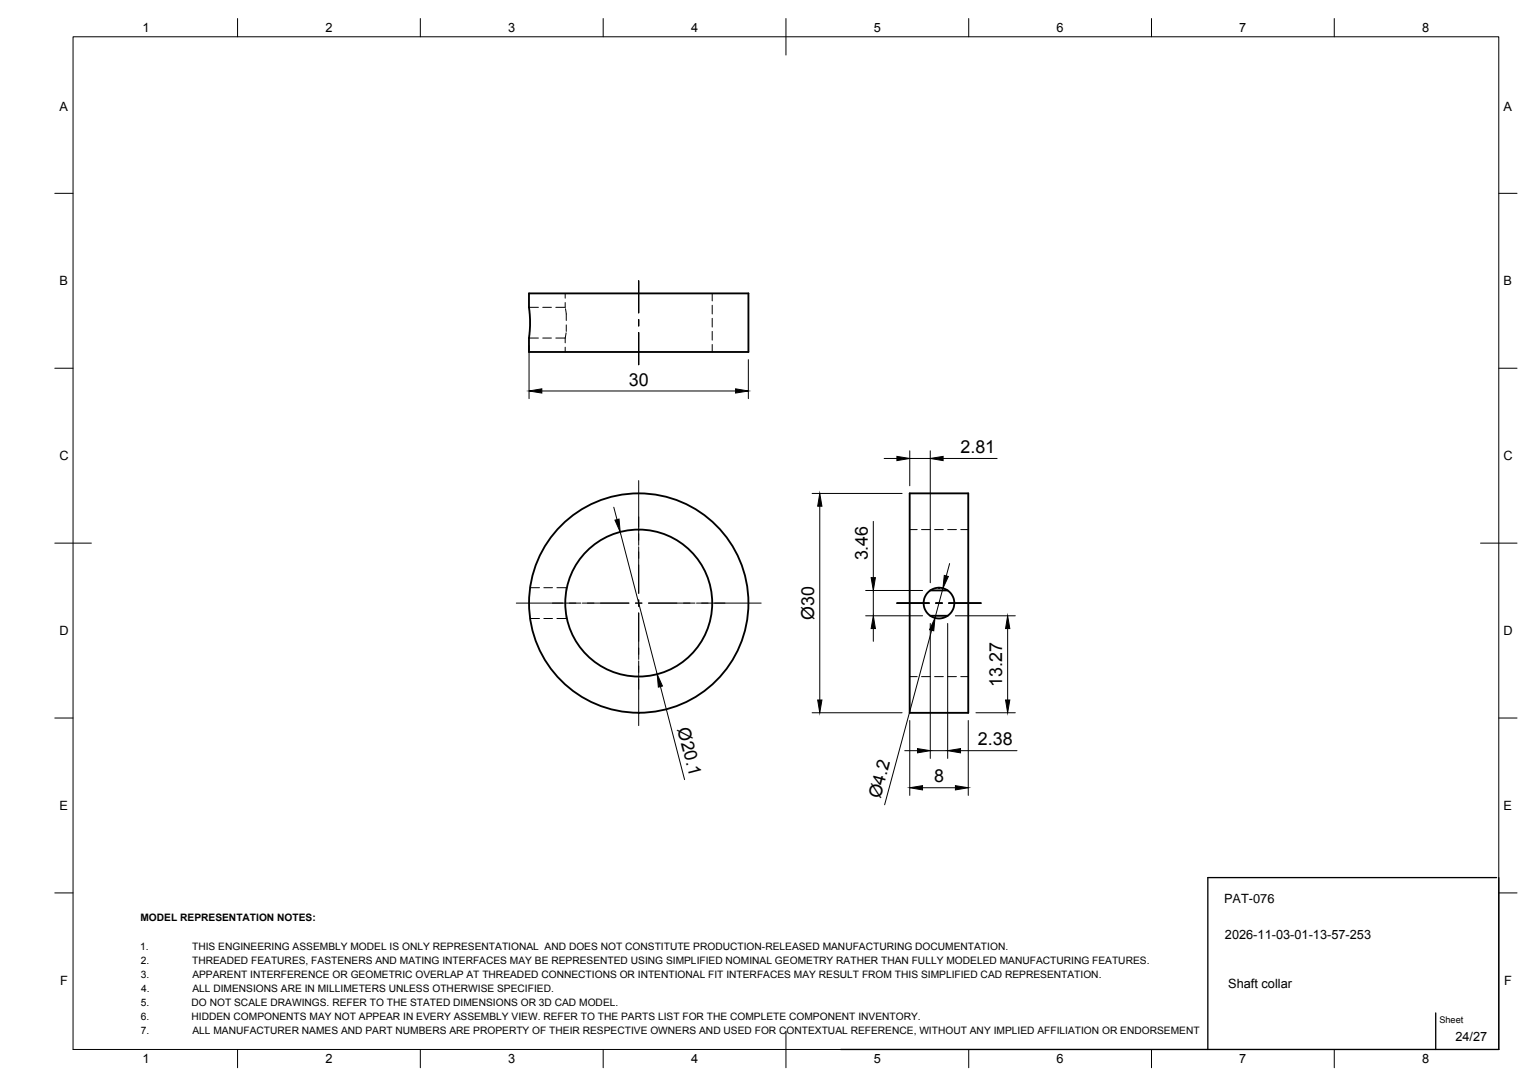
ISO-10303-21;
HEADER;
/* Generated by software containing ST-Developer
 * from STEP Tools, Inc. (www.steptools.com) 
 */

FILE_DESCRIPTION(
/* description */ ('Overhung pulley bearing cartridge'),
/* implementation_level */ '2;1');

FILE_NAME(
/* name */ 'Shaft collar.step',
/* time_stamp */ '2026-10-28T03:22:33-07:00',
/* author */ (''),
/* organization */ (''),
/* preprocessor_version */ 'ST-DEVELOPER v20.2',
/* originating_system */ 'Autodesk Translation Framework v15.17.0.0',
/* authorisation */ '');

FILE_SCHEMA (('AUTOMOTIVE_DESIGN { 1 0 10303 214 3 1 1 }'));
ENDSEC;

DATA;
#10=MECHANICAL_DESIGN_GEOMETRIC_PRESENTATION_REPRESENTATION('',(#308),#10963);
#181=B_SPLINE_CURVE_WITH_KNOTS('',3,(#9804,#9805,#9806,#9807,#9808,#9809,
#9810,#9811,#9812,#9813,#9814,#9815,#9816,#9817),.UNSPECIFIED.,.F.,.F.,
(4,2,2,2,2,2,4),(0.756005737987012,0.793568827564648,0.872922520054202,
0.952276212543757,1.03162990503331,1.11098359752287,1.1485466871005),
 .UNSPECIFIED.);
#182=B_SPLINE_CURVE_WITH_KNOTS('',3,(#9823,#9824,#9825,#9826,#9827,#9828,
#9829,#9830,#9831,#9832,#9833,#9834,#9835,#9836,#9837,#9838,#9839,#9840),
 .UNSPECIFIED.,.F.,.F.,(4,2,2,2,2,2,2,2,4),(0.,0.0792165807733632,0.158433161546726,
0.237648697074571,0.316864232602415,0.396079768130259,0.475295303658103,
0.554511884431466,0.63372846520483),.UNSPECIFIED.);
#183=B_SPLINE_CURVE_WITH_KNOTS('',3,(#9841,#9842,#9843,#9844,#9845,#9846,
#9847,#9848,#9849,#9850,#9851,#9852,#9853,#9854,#9855,#9856,#9857,#9858),
 .UNSPECIFIED.,.F.,.F.,(4,2,2,2,2,2,2,2,4),(0.63372846520483,0.712945045978192,
0.792161626751555,0.8713771622794,0.950592697807244,1.02980823333509,1.10902376886293,
1.1882403496363,1.26745693040966),.UNSPECIFIED.);
#184=B_SPLINE_CURVE_WITH_KNOTS('',3,(#9861,#9862,#9863,#9864,#9865,#9866,
#9867,#9868,#9869,#9870,#9871,#9872,#9873,#9874),.UNSPECIFIED.,.F.,.F.,
(4,2,2,2,2,2,4),(0.121154929624506,0.158718019202143,0.238071711691698,
0.317425404181252,0.396779096670807,0.476132789160362,0.513695878738),
 .UNSPECIFIED.);
#256=SHAPE_REPRESENTATION_RELATIONSHIP('SRR','None',#11078,#278);
#278=ADVANCED_BREP_SHAPE_REPRESENTATION('',(#336),#10958);
#308=STYLED_ITEM('',(#11253),#336);
#336=MANIFOLD_SOLID_BREP('Body1',#5677);
#413=FACE_BOUND('',#1179,.T.);
#414=FACE_BOUND('',#1181,.T.);
#415=FACE_BOUND('',#1183,.T.);
#416=FACE_BOUND('',#1185,.T.);
#542=PLANE('',#6355);
#543=PLANE('',#6360);
#544=PLANE('',#6367);
#545=PLANE('',#6368);
#774=FACE_OUTER_BOUND('',#1175,.T.);
#775=FACE_OUTER_BOUND('',#1176,.T.);
#776=FACE_OUTER_BOUND('',#1177,.T.);
#777=FACE_OUTER_BOUND('',#1178,.T.);
#778=FACE_OUTER_BOUND('',#1180,.T.);
#779=FACE_OUTER_BOUND('',#1182,.T.);
#780=FACE_OUTER_BOUND('',#1184,.T.);
#1175=EDGE_LOOP('',(#4435,#4436));
#1176=EDGE_LOOP('',(#4437,#4438,#4439,#4440,#4441,#4442,#4443,#4444,#4445));
#1177=EDGE_LOOP('',(#4446,#4447,#4448));
#1178=EDGE_LOOP('',(#4449,#4450,#4451,#4452));
#1179=EDGE_LOOP('',(#4453,#4454,#4455,#4456));
#1180=EDGE_LOOP('',(#4457,#4458,#4459,#4460));
#1181=EDGE_LOOP('',(#4461,#4462));
#1182=EDGE_LOOP('',(#4463));
#1183=EDGE_LOOP('',(#4464));
#1184=EDGE_LOOP('',(#4465));
#1185=EDGE_LOOP('',(#4466));
#1517=LINE('',#9800,#1859);
#1518=LINE('',#9821,#1860);
#1519=LINE('',#9876,#1861);
#1520=LINE('',#9881,#1862);
#1521=LINE('',#9887,#1863);
#1859=VECTOR('',#7739,1.);
#1860=VECTOR('',#7746,0.21);
#1861=VECTOR('',#7751,1.);
#1862=VECTOR('',#7756,1.005);
#1863=VECTOR('',#7763,1.5);
#2196=CIRCLE('',#6356,0.21);
#2197=CIRCLE('',#6358,0.21);
#2198=CIRCLE('',#6359,0.21);
#2199=CIRCLE('',#6362,1.005);
#2200=CIRCLE('',#6363,1.005);
#2201=CIRCLE('',#6365,1.5);
#2202=CIRCLE('',#6366,1.5);
#2649=VERTEX_POINT('',#9798);
#2650=VERTEX_POINT('',#9799);
#2651=VERTEX_POINT('',#9803);
#2652=VERTEX_POINT('',#9818);
#2653=VERTEX_POINT('',#9820);
#2654=VERTEX_POINT('',#9822);
#2655=VERTEX_POINT('',#9859);
#2656=VERTEX_POINT('',#9878);
#2657=VERTEX_POINT('',#9880);
#2658=VERTEX_POINT('',#9884);
#2659=VERTEX_POINT('',#9886);
#3287=EDGE_CURVE('',#2649,#2650,#1517,.T.);
#3288=EDGE_CURVE('',#2649,#2650,#2196,.T.);
#3289=EDGE_CURVE('',#2651,#2649,#181,.T.);
#3290=EDGE_CURVE('',#2652,#2651,#2197,.T.);
#3291=EDGE_CURVE('',#2652,#2653,#1518,.T.);
#3292=EDGE_CURVE('',#2654,#2653,#182,.T.);
#3293=EDGE_CURVE('',#2653,#2654,#183,.T.);
#3294=EDGE_CURVE('',#2655,#2652,#2198,.T.);
#3295=EDGE_CURVE('',#2650,#2655,#184,.T.);
#3296=EDGE_CURVE('',#2655,#2651,#1519,.T.);
#3297=EDGE_CURVE('',#2656,#2656,#2199,.T.);
#3298=EDGE_CURVE('',#2656,#2657,#1520,.T.);
#3299=EDGE_CURVE('',#2657,#2657,#2200,.T.);
#3300=EDGE_CURVE('',#2658,#2658,#2201,.T.);
#3301=EDGE_CURVE('',#2658,#2659,#1521,.T.);
#3302=EDGE_CURVE('',#2659,#2659,#2202,.T.);
#4435=ORIENTED_EDGE('',*,*,#3287,.F.);
#4436=ORIENTED_EDGE('',*,*,#3288,.T.);
#4437=ORIENTED_EDGE('',*,*,#3289,.F.);
#4438=ORIENTED_EDGE('',*,*,#3290,.F.);
#4439=ORIENTED_EDGE('',*,*,#3291,.T.);
#4440=ORIENTED_EDGE('',*,*,#3292,.F.);
#4441=ORIENTED_EDGE('',*,*,#3293,.F.);
#4442=ORIENTED_EDGE('',*,*,#3291,.F.);
#4443=ORIENTED_EDGE('',*,*,#3294,.F.);
#4444=ORIENTED_EDGE('',*,*,#3295,.F.);
#4445=ORIENTED_EDGE('',*,*,#3288,.F.);
#4446=ORIENTED_EDGE('',*,*,#3296,.F.);
#4447=ORIENTED_EDGE('',*,*,#3294,.T.);
#4448=ORIENTED_EDGE('',*,*,#3290,.T.);
#4449=ORIENTED_EDGE('',*,*,#3297,.F.);
#4450=ORIENTED_EDGE('',*,*,#3298,.T.);
#4451=ORIENTED_EDGE('',*,*,#3299,.T.);
#4452=ORIENTED_EDGE('',*,*,#3298,.F.);
#4453=ORIENTED_EDGE('',*,*,#3295,.T.);
#4454=ORIENTED_EDGE('',*,*,#3296,.T.);
#4455=ORIENTED_EDGE('',*,*,#3289,.T.);
#4456=ORIENTED_EDGE('',*,*,#3287,.T.);
#4457=ORIENTED_EDGE('',*,*,#3300,.F.);
#4458=ORIENTED_EDGE('',*,*,#3301,.T.);
#4459=ORIENTED_EDGE('',*,*,#3302,.T.);
#4460=ORIENTED_EDGE('',*,*,#3301,.F.);
#4461=ORIENTED_EDGE('',*,*,#3292,.T.);
#4462=ORIENTED_EDGE('',*,*,#3293,.T.);
#4463=ORIENTED_EDGE('',*,*,#3300,.T.);
#4464=ORIENTED_EDGE('',*,*,#3297,.T.);
#4465=ORIENTED_EDGE('',*,*,#3302,.F.);
#4466=ORIENTED_EDGE('',*,*,#3299,.F.);
#5226=CYLINDRICAL_SURFACE('',#6357,0.21);
#5227=CYLINDRICAL_SURFACE('',#6361,1.005);
#5228=CYLINDRICAL_SURFACE('',#6364,1.5);
#5518=ADVANCED_FACE('',(#774),#542,.T.);
#5519=ADVANCED_FACE('',(#775),#5226,.F.);
#5520=ADVANCED_FACE('',(#776),#543,.T.);
#5521=ADVANCED_FACE('',(#777,#413),#5227,.F.);
#5522=ADVANCED_FACE('',(#778,#414),#5228,.T.);
#5523=ADVANCED_FACE('',(#779,#415),#544,.T.);
#5524=ADVANCED_FACE('',(#780,#416),#545,.F.);
#5677=CLOSED_SHELL('',(#5518,#5519,#5520,#5521,#5522,#5523,#5524));
#6354=AXIS2_PLACEMENT_3D('',#9796,#7735,#7736);
#6355=AXIS2_PLACEMENT_3D('',#9797,#7737,#7738);
#6356=AXIS2_PLACEMENT_3D('',#9801,#7740,#7741);
#6357=AXIS2_PLACEMENT_3D('',#9802,#7742,#7743);
#6358=AXIS2_PLACEMENT_3D('',#9819,#7744,#7745);
#6359=AXIS2_PLACEMENT_3D('',#9860,#7747,#7748);
#6360=AXIS2_PLACEMENT_3D('',#9875,#7749,#7750);
#6361=AXIS2_PLACEMENT_3D('',#9877,#7752,#7753);
#6362=AXIS2_PLACEMENT_3D('',#9879,#7754,#7755);
#6363=AXIS2_PLACEMENT_3D('',#9882,#7757,#7758);
#6364=AXIS2_PLACEMENT_3D('',#9883,#7759,#7760);
#6365=AXIS2_PLACEMENT_3D('',#9885,#7761,#7762);
#6366=AXIS2_PLACEMENT_3D('',#9888,#7764,#7765);
#6367=AXIS2_PLACEMENT_3D('',#9889,#7766,#7767);
#6368=AXIS2_PLACEMENT_3D('',#9890,#7768,#7769);
#7735=DIRECTION('axis',(0.,0.,1.));
#7736=DIRECTION('refdir',(1.,0.,0.));
#7737=DIRECTION('center_axis',(0.,0.,1.));
#7738=DIRECTION('ref_axis',(1.,0.,0.));
#7739=DIRECTION('',(0.,1.,0.));
#7740=DIRECTION('center_axis',(0.,0.,1.));
#7741=DIRECTION('ref_axis',(1.,0.,0.));
#7742=DIRECTION('center_axis',(0.,0.,1.));
#7743=DIRECTION('ref_axis',(1.,0.,0.));
#7744=DIRECTION('center_axis',(0.,0.,1.));
#7745=DIRECTION('ref_axis',(1.,0.,0.));
#7746=DIRECTION('',(0.,0.,1.));
#7747=DIRECTION('center_axis',(0.,0.,1.));
#7748=DIRECTION('ref_axis',(1.,0.,0.));
#7749=DIRECTION('center_axis',(0.,0.,1.));
#7750=DIRECTION('ref_axis',(1.,0.,0.));
#7751=DIRECTION('',(0.,-1.,0.));
#7752=DIRECTION('center_axis',(0.,1.,0.));
#7753=DIRECTION('ref_axis',(1.,0.,0.));
#7754=DIRECTION('center_axis',(0.,-1.,0.));
#7755=DIRECTION('ref_axis',(1.,0.,0.));
#7756=DIRECTION('',(0.,-1.,0.));
#7757=DIRECTION('center_axis',(0.,-1.,0.));
#7758=DIRECTION('ref_axis',(1.,0.,0.));
#7759=DIRECTION('center_axis',(0.,1.,0.));
#7760=DIRECTION('ref_axis',(1.,0.,0.));
#7761=DIRECTION('center_axis',(0.,1.,0.));
#7762=DIRECTION('ref_axis',(1.,0.,0.));
#7763=DIRECTION('',(0.,-1.,0.));
#7764=DIRECTION('center_axis',(0.,1.,0.));
#7765=DIRECTION('ref_axis',(1.,0.,0.));
#7766=DIRECTION('center_axis',(0.,1.,0.));
#7767=DIRECTION('ref_axis',(1.,0.,0.));
#7768=DIRECTION('center_axis',(0.,1.,0.));
#7769=DIRECTION('ref_axis',(1.,0.,0.));
#9796=CARTESIAN_POINT('',(0.,0.,0.));
#9797=CARTESIAN_POINT('Origin',(0.,6.8,5.49));
#9798=CARTESIAN_POINT('',(0.172988438920061,6.68094119100209,5.49));
#9799=CARTESIAN_POINT('',(0.172988438920061,6.91905880899791,5.49));
#9800=CARTESIAN_POINT('',(0.172988438920061,6.4,5.49));
#9801=CARTESIAN_POINT('Origin',(0.,6.8,5.49));
#9802=CARTESIAN_POINT('Origin',(0.,6.8,5.49));
#9803=CARTESIAN_POINT('',(-0.172988438920061,6.68094119100209,5.49));
#9804=CARTESIAN_POINT('Ctrl Pts',(-0.172988438920061,6.68094119100209,5.49));
#9805=CARTESIAN_POINT('Ctrl Pts',(-0.165594865311318,6.67019857760471,5.49129192197638));
#9806=CARTESIAN_POINT('Ctrl Pts',(-0.157297138725608,6.66031229062726,5.49265394943905));
#9807=CARTESIAN_POINT('Ctrl Pts',(-0.129892073845076,6.63290722574673,5.4967480843909));
#9808=CARTESIAN_POINT('Ctrl Pts',(-0.106330167759285,6.61675794366705,5.49969589327638));
#9809=CARTESIAN_POINT('Ctrl Pts',(-0.0546129046324107,6.59530220603509,
5.50385029472357));
#9810=CARTESIAN_POINT('Ctrl Pts',(-0.0264512308298516,6.59,5.505));
#9811=CARTESIAN_POINT('Ctrl Pts',(0.0264512308298515,6.59,5.505));
#9812=CARTESIAN_POINT('Ctrl Pts',(0.0546129046324106,6.59530220603509,5.50385029472357));
#9813=CARTESIAN_POINT('Ctrl Pts',(0.106330167759285,6.61675794366705,5.49969589327638));
#9814=CARTESIAN_POINT('Ctrl Pts',(0.129892073845076,6.63290722574673,5.4967480843909));
#9815=CARTESIAN_POINT('Ctrl Pts',(0.157297138725608,6.66031229062726,5.49265394943905));
#9816=CARTESIAN_POINT('Ctrl Pts',(0.165594865311318,6.67019857760471,5.49129192197638));
#9817=CARTESIAN_POINT('Ctrl Pts',(0.172988438920061,6.68094119100209,5.49));
#9818=CARTESIAN_POINT('',(-0.21,6.8,5.49));
#9819=CARTESIAN_POINT('Origin',(0.,6.8,5.49));
#9820=CARTESIAN_POINT('',(-0.21,6.8,5.98522725533839));
#9821=CARTESIAN_POINT('',(-0.21,6.8,5.49));
#9822=CARTESIAN_POINT('',(0.21,6.8,5.98522725533839));
#9823=CARTESIAN_POINT('Ctrl Pts',(0.21,6.8,5.98522725533839));
#9824=CARTESIAN_POINT('Ctrl Pts',(0.21,6.77359447307555,5.98522725533839));
#9825=CARTESIAN_POINT('Ctrl Pts',(0.204715737269596,6.74545292590929,5.98600415954412));
#9826=CARTESIAN_POINT('Ctrl Pts',(0.183273763036331,6.69372373109487,5.98880073282317));
#9827=CARTESIAN_POINT('Ctrl Pts',(0.167117923970394,6.67013307587204,5.99077897157582));
#9828=CARTESIAN_POINT('Ctrl Pts',(0.129867169887369,6.63288232178902,5.99448481141327));
#9829=CARTESIAN_POINT('Ctrl Pts',(0.106276408305765,6.61672628999865,5.99645455657129));
#9830=CARTESIAN_POINT('Ctrl Pts',(0.0545468514059003,6.59528417517378,5.99923165515646));
#9831=CARTESIAN_POINT('Ctrl Pts',(0.0264051785092814,6.59,6.));
#9832=CARTESIAN_POINT('Ctrl Pts',(-0.0264051785092814,6.59,6.));
#9833=CARTESIAN_POINT('Ctrl Pts',(-0.0545468514059002,6.59528417517378,
5.99923165515646));
#9834=CARTESIAN_POINT('Ctrl Pts',(-0.106276408305765,6.61672628999865,5.99645455657129));
#9835=CARTESIAN_POINT('Ctrl Pts',(-0.129867169887369,6.63288232178902,5.99448481141327));
#9836=CARTESIAN_POINT('Ctrl Pts',(-0.167117923970394,6.67013307587204,5.99077897157582));
#9837=CARTESIAN_POINT('Ctrl Pts',(-0.183273763036331,6.69372373109487,5.98880073282317));
#9838=CARTESIAN_POINT('Ctrl Pts',(-0.204715737269596,6.74545292590929,5.98600415954412));
#9839=CARTESIAN_POINT('Ctrl Pts',(-0.21,6.77359447307555,5.98522725533839));
#9840=CARTESIAN_POINT('Ctrl Pts',(-0.21,6.8,5.98522725533839));
#9841=CARTESIAN_POINT('Ctrl Pts',(-0.21,6.8,5.98522725533839));
#9842=CARTESIAN_POINT('Ctrl Pts',(-0.21,6.82640552692445,5.98522725533839));
#9843=CARTESIAN_POINT('Ctrl Pts',(-0.204715737269596,6.85454707409071,5.98600415954412));
#9844=CARTESIAN_POINT('Ctrl Pts',(-0.183273763036331,6.90627626890513,5.98880073282317));
#9845=CARTESIAN_POINT('Ctrl Pts',(-0.167117923970394,6.92986692412796,5.99077897157582));
#9846=CARTESIAN_POINT('Ctrl Pts',(-0.129867169887369,6.96711767821098,5.99448481141327));
#9847=CARTESIAN_POINT('Ctrl Pts',(-0.106276408305765,6.98327371000135,5.99645455657129));
#9848=CARTESIAN_POINT('Ctrl Pts',(-0.0545468514059003,7.00471582482622,
5.99923165515646));
#9849=CARTESIAN_POINT('Ctrl Pts',(-0.0264051785092815,7.01,6.));
#9850=CARTESIAN_POINT('Ctrl Pts',(0.0264051785092814,7.01,6.));
#9851=CARTESIAN_POINT('Ctrl Pts',(0.0545468514058999,7.00471582482622,5.99923165515646));
#9852=CARTESIAN_POINT('Ctrl Pts',(0.106276408305765,6.98327371000135,5.99645455657129));
#9853=CARTESIAN_POINT('Ctrl Pts',(0.129867169887369,6.96711767821098,5.99448481141327));
#9854=CARTESIAN_POINT('Ctrl Pts',(0.167117923970393,6.92986692412796,5.99077897157582));
#9855=CARTESIAN_POINT('Ctrl Pts',(0.183273763036332,6.90627626890513,5.98880073282317));
#9856=CARTESIAN_POINT('Ctrl Pts',(0.204715737269596,6.85454707409071,5.98600415954412));
#9857=CARTESIAN_POINT('Ctrl Pts',(0.21,6.82640552692445,5.98522725533839));
#9858=CARTESIAN_POINT('Ctrl Pts',(0.21,6.8,5.98522725533839));
#9859=CARTESIAN_POINT('',(-0.172988438920061,6.91905880899791,5.49));
#9860=CARTESIAN_POINT('Origin',(0.,6.8,5.49));
#9861=CARTESIAN_POINT('Ctrl Pts',(0.172988438920062,6.91905880899791,5.49));
#9862=CARTESIAN_POINT('Ctrl Pts',(0.165594865311319,6.92980142239529,5.49129192197638));
#9863=CARTESIAN_POINT('Ctrl Pts',(0.157297138725609,6.93968770937274,5.49265394943905));
#9864=CARTESIAN_POINT('Ctrl Pts',(0.129892073845076,6.96709277425327,5.4967480843909));
#9865=CARTESIAN_POINT('Ctrl Pts',(0.106330167759285,6.98324205633295,5.49969589327638));
#9866=CARTESIAN_POINT('Ctrl Pts',(0.0546129046324107,7.00469779396491,5.50385029472357));
#9867=CARTESIAN_POINT('Ctrl Pts',(0.0264512308298516,7.01,5.505));
#9868=CARTESIAN_POINT('Ctrl Pts',(-0.0264512308298515,7.01,5.505));
#9869=CARTESIAN_POINT('Ctrl Pts',(-0.0546129046324097,7.00469779396491,
5.50385029472357));
#9870=CARTESIAN_POINT('Ctrl Pts',(-0.106330167759284,6.98324205633295,5.49969589327638));
#9871=CARTESIAN_POINT('Ctrl Pts',(-0.129892073845076,6.96709277425327,5.4967480843909));
#9872=CARTESIAN_POINT('Ctrl Pts',(-0.157297138725609,6.93968770937274,5.49265394943905));
#9873=CARTESIAN_POINT('Ctrl Pts',(-0.165594865311318,6.92980142239529,5.49129192197638));
#9874=CARTESIAN_POINT('Ctrl Pts',(-0.172988438920061,6.91905880899791,5.49));
#9875=CARTESIAN_POINT('Origin',(0.,6.8,5.49));
#9876=CARTESIAN_POINT('',(-0.172988438920061,6.4,5.49));
#9877=CARTESIAN_POINT('Origin',(0.,6.4,4.5));
#9878=CARTESIAN_POINT('',(-1.005,7.2,4.5));
#9879=CARTESIAN_POINT('Origin',(0.,7.2,4.5));
#9880=CARTESIAN_POINT('',(-1.005,6.4,4.5));
#9881=CARTESIAN_POINT('',(-1.005,6.4,4.5));
#9882=CARTESIAN_POINT('Origin',(0.,6.4,4.5));
#9883=CARTESIAN_POINT('Origin',(0.,6.4,4.5));
#9884=CARTESIAN_POINT('',(-1.5,7.2,4.5));
#9885=CARTESIAN_POINT('Origin',(0.,7.2,4.5));
#9886=CARTESIAN_POINT('',(-1.5,6.4,4.5));
#9887=CARTESIAN_POINT('',(-1.5,6.4,4.5));
#9888=CARTESIAN_POINT('Origin',(0.,6.4,4.5));
#9889=CARTESIAN_POINT('Origin',(0.,7.2,4.5));
#9890=CARTESIAN_POINT('Origin',(0.,6.4,4.5));
#10931=UNCERTAINTY_MEASURE_WITH_UNIT(LENGTH_MEASURE(0.001),#10964,
'DISTANCE_ACCURACY_VALUE',
'Maximum model space distance between geometric entities at asserted c
onnectivities');
#10936=UNCERTAINTY_MEASURE_WITH_UNIT(LENGTH_MEASURE(0.001),#10964,
'DISTANCE_ACCURACY_VALUE',
'Maximum model space distance between geometric entities at asserted c
onnectivities');
#10958=(
GEOMETRIC_REPRESENTATION_CONTEXT(3)
GLOBAL_UNCERTAINTY_ASSIGNED_CONTEXT((#10931))
GLOBAL_UNIT_ASSIGNED_CONTEXT((#10964,#10966,#10967))
REPRESENTATION_CONTEXT('','3D')
);
#10963=(
GEOMETRIC_REPRESENTATION_CONTEXT(3)
GLOBAL_UNCERTAINTY_ASSIGNED_CONTEXT((#10936))
GLOBAL_UNIT_ASSIGNED_CONTEXT((#10964,#10966,#10967))
REPRESENTATION_CONTEXT('','3D')
);
#10964=(
LENGTH_UNIT()
NAMED_UNIT(*)
SI_UNIT(.CENTI.,.METRE.)
);
#10966=(
NAMED_UNIT(*)
PLANE_ANGLE_UNIT()
SI_UNIT($,.RADIAN.)
);
#10967=(
NAMED_UNIT(*)
SI_UNIT($,.STERADIAN.)
SOLID_ANGLE_UNIT()
);
#10989=SHAPE_DEFINITION_REPRESENTATION(#11042,#11078);
#11042=PRODUCT_DEFINITION_SHAPE('',$,#11105);
#11078=SHAPE_REPRESENTATION('',(#6354),#10958);
#11083=PRODUCT_DEFINITION_CONTEXT('part definition',#11163,'design');
#11105=PRODUCT_DEFINITION('Shaft collar','Shaft collar',#11131,#11083);
#11131=PRODUCT_DEFINITION_FORMATION('',$,#11186);
#11163=APPLICATION_CONTEXT(
'Core Data for Automotive Mechanical Design Process');
#11164=PRODUCT_CONTEXT('part definition',#11163,'mechanical');
#11186=PRODUCT('Shaft collar','Shaft collar','Shaft collar',(#11164));
#11247=COLOUR_RGB('Grey',0.48,0.52,0.57);
#11248=FILL_AREA_STYLE_COLOUR('',#11247);
#11249=FILL_AREA_STYLE('',(#11248));
#11250=SURFACE_STYLE_FILL_AREA(#11249);
#11251=SURFACE_SIDE_STYLE('',(#11250));
#11252=SURFACE_STYLE_USAGE(.BOTH.,#11251);
#11253=PRESENTATION_STYLE_ASSIGNMENT((#11252));
ENDSEC;
END-ISO-10303-21;
